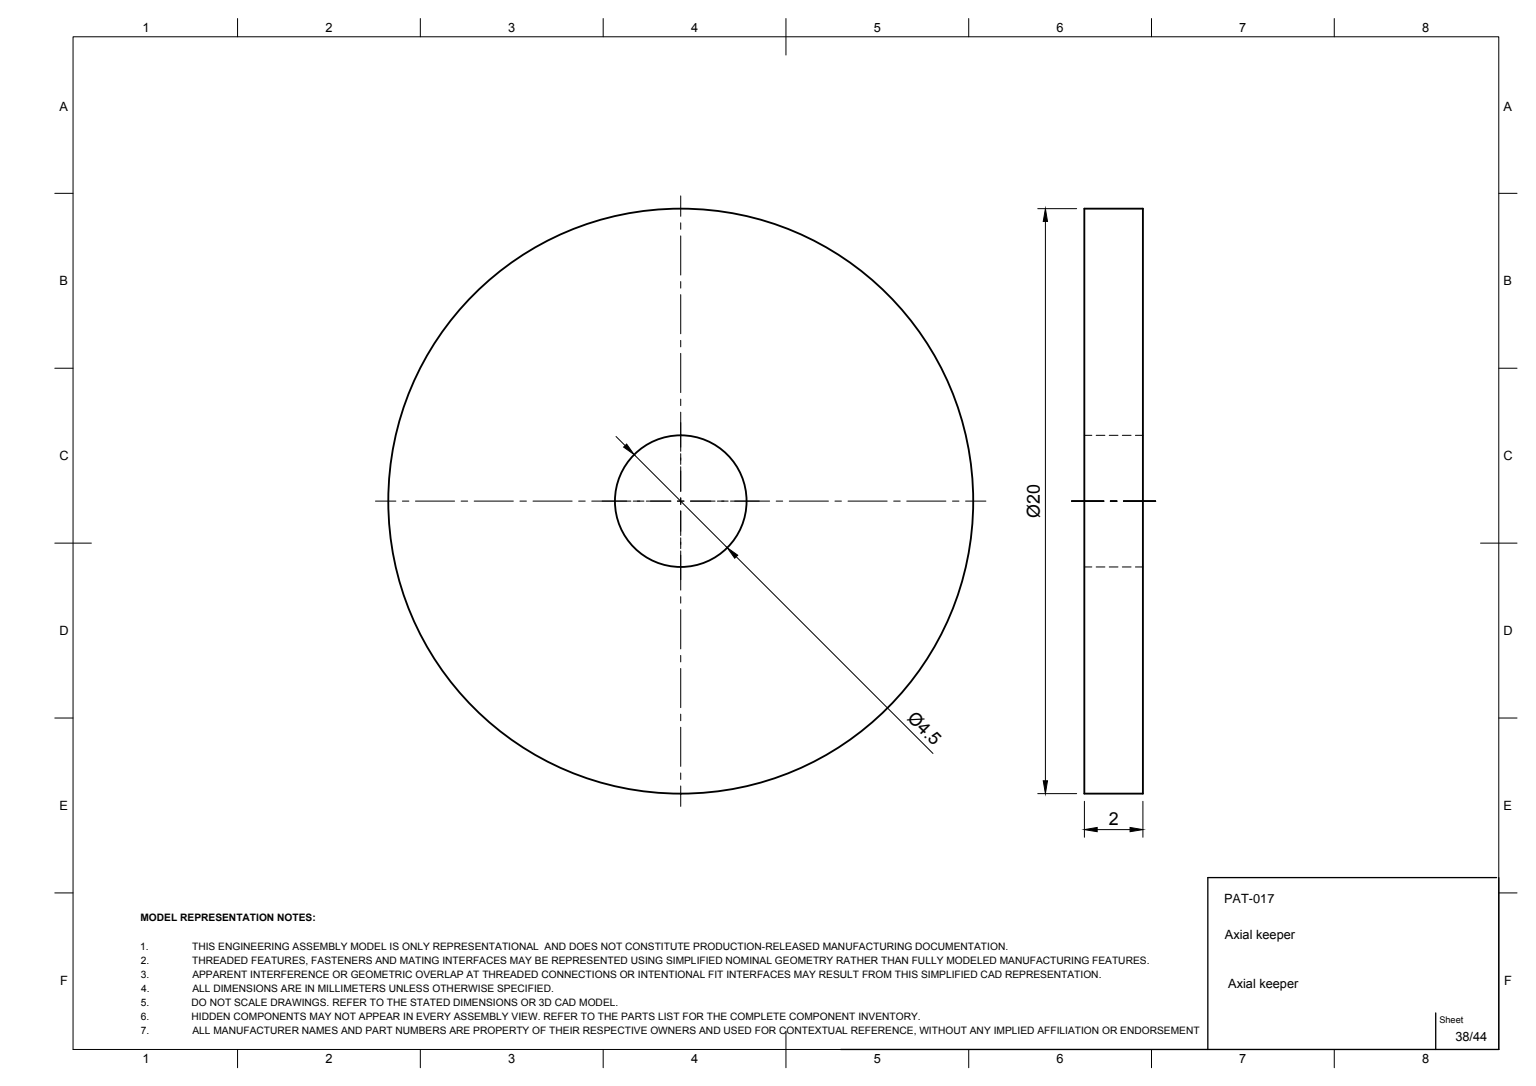
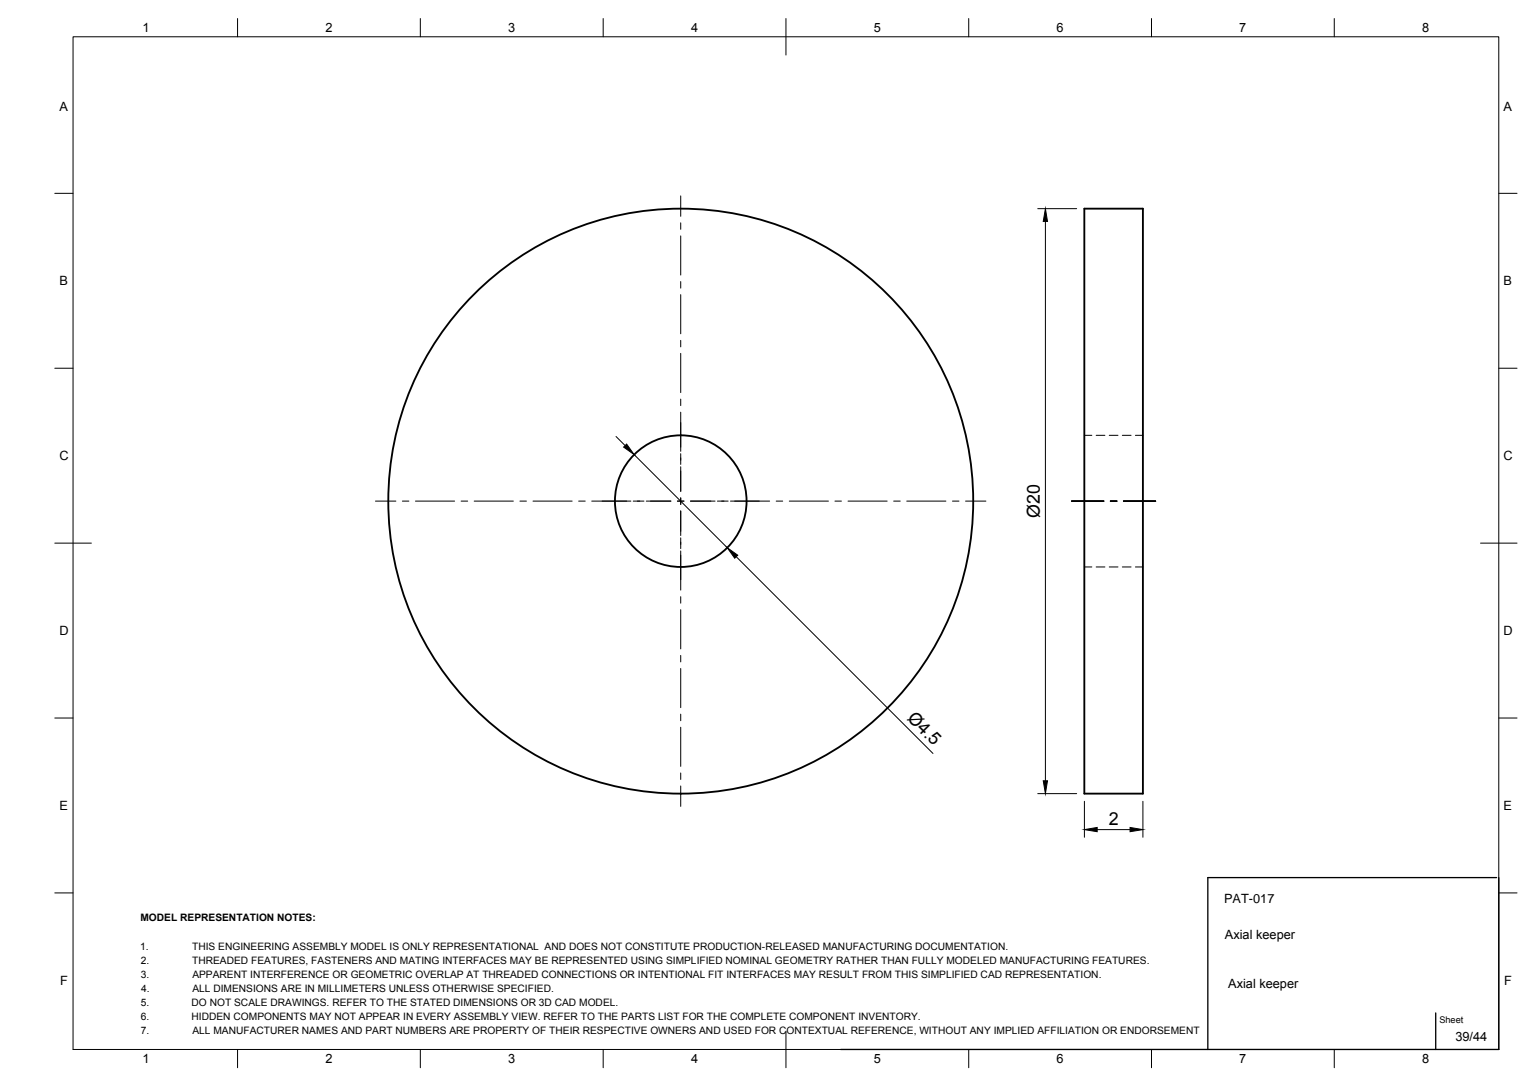
ISO-10303-21;
HEADER;
/* Generated by software containing ST-Developer
 * from STEP Tools, Inc. (www.steptools.com) 
 */

FILE_DESCRIPTION(
/* description */ ('Cam-and-follower valve demonstrator'),
/* implementation_level */ '2;1');

FILE_NAME(
/* name */ 'Axial keeper.step',
/* time_stamp */ '2026-10-28T03:25:17-07:00',
/* author */ (''),
/* organization */ (''),
/* preprocessor_version */ 'ST-DEVELOPER v20.2',
/* originating_system */ 'Autodesk Translation Framework v15.17.0.0',
/* authorisation */ '');

FILE_SCHEMA (('AUTOMOTIVE_DESIGN { 1 0 10303 214 3 1 1 }'));
ENDSEC;

DATA;
#10=MECHANICAL_DESIGN_GEOMETRIC_PRESENTATION_REPRESENTATION('',(#448),#12896);
#369=SHAPE_REPRESENTATION_RELATIONSHIP('SRR','None',#13088,#405);
#405=ADVANCED_BREP_SHAPE_REPRESENTATION('',(#489),#12888);
#448=STYLED_ITEM('',(#13316),#489);
#489=MANIFOLD_SOLID_BREP('Body1',#6217);
#648=FACE_BOUND('',#1934,.T.);
#649=FACE_BOUND('',#1936,.T.);
#945=CIRCLE('',#7265,0.225);
#946=CIRCLE('',#7266,0.225);
#947=CIRCLE('',#7268,1.);
#948=CIRCLE('',#7269,1.);
#1083=CYLINDRICAL_SURFACE('',#7264,0.225);
#1084=CYLINDRICAL_SURFACE('',#7267,1.);
#1410=FACE_OUTER_BOUND('',#1931,.T.);
#1411=FACE_OUTER_BOUND('',#1932,.T.);
#1412=FACE_OUTER_BOUND('',#1933,.T.);
#1413=FACE_OUTER_BOUND('',#1935,.T.);
#1931=EDGE_LOOP('',(#5401,#5402,#5403,#5404));
#1932=EDGE_LOOP('',(#5405,#5406,#5407,#5408));
#1933=EDGE_LOOP('',(#5409));
#1934=EDGE_LOOP('',(#5410));
#1935=EDGE_LOOP('',(#5411));
#1936=EDGE_LOOP('',(#5412));
#2347=LINE('',#12531,#2769);
#2348=LINE('',#12537,#2770);
#2769=VECTOR('',#9054,0.225);
#2770=VECTOR('',#9061,1.);
#3280=VERTEX_POINT('',#12528);
#3281=VERTEX_POINT('',#12530);
#3282=VERTEX_POINT('',#12534);
#3283=VERTEX_POINT('',#12536);
#3997=EDGE_CURVE('',#3280,#3280,#945,.T.);
#3998=EDGE_CURVE('',#3280,#3281,#2347,.T.);
#3999=EDGE_CURVE('',#3281,#3281,#946,.T.);
#4000=EDGE_CURVE('',#3282,#3282,#947,.T.);
#4001=EDGE_CURVE('',#3282,#3283,#2348,.T.);
#4002=EDGE_CURVE('',#3283,#3283,#948,.T.);
#5401=ORIENTED_EDGE('',*,*,#3997,.F.);
#5402=ORIENTED_EDGE('',*,*,#3998,.T.);
#5403=ORIENTED_EDGE('',*,*,#3999,.T.);
#5404=ORIENTED_EDGE('',*,*,#3998,.F.);
#5405=ORIENTED_EDGE('',*,*,#4000,.F.);
#5406=ORIENTED_EDGE('',*,*,#4001,.T.);
#5407=ORIENTED_EDGE('',*,*,#4002,.T.);
#5408=ORIENTED_EDGE('',*,*,#4001,.F.);
#5409=ORIENTED_EDGE('',*,*,#4000,.T.);
#5410=ORIENTED_EDGE('',*,*,#3997,.T.);
#5411=ORIENTED_EDGE('',*,*,#4002,.F.);
#5412=ORIENTED_EDGE('',*,*,#3999,.F.);
#5774=PLANE('',#7270);
#5775=PLANE('',#7271);
#6126=ADVANCED_FACE('',(#1410),#1083,.F.);
#6127=ADVANCED_FACE('',(#1411),#1084,.T.);
#6128=ADVANCED_FACE('',(#1412,#648),#5774,.T.);
#6129=ADVANCED_FACE('',(#1413,#649),#5775,.F.);
#6217=CLOSED_SHELL('',(#6126,#6127,#6128,#6129));
#7263=AXIS2_PLACEMENT_3D('',#12526,#9048,#9049);
#7264=AXIS2_PLACEMENT_3D('',#12527,#9050,#9051);
#7265=AXIS2_PLACEMENT_3D('',#12529,#9052,#9053);
#7266=AXIS2_PLACEMENT_3D('',#12532,#9055,#9056);
#7267=AXIS2_PLACEMENT_3D('',#12533,#9057,#9058);
#7268=AXIS2_PLACEMENT_3D('',#12535,#9059,#9060);
#7269=AXIS2_PLACEMENT_3D('',#12538,#9062,#9063);
#7270=AXIS2_PLACEMENT_3D('',#12539,#9064,#9065);
#7271=AXIS2_PLACEMENT_3D('',#12540,#9066,#9067);
#9048=DIRECTION('axis',(0.,0.,1.));
#9049=DIRECTION('refdir',(1.,0.,0.));
#9050=DIRECTION('center_axis',(0.,1.,0.));
#9051=DIRECTION('ref_axis',(1.,0.,0.));
#9052=DIRECTION('center_axis',(0.,-1.,0.));
#9053=DIRECTION('ref_axis',(1.,0.,0.));
#9054=DIRECTION('',(0.,-1.,0.));
#9055=DIRECTION('center_axis',(0.,-1.,0.));
#9056=DIRECTION('ref_axis',(1.,0.,0.));
#9057=DIRECTION('center_axis',(0.,1.,0.));
#9058=DIRECTION('ref_axis',(1.,0.,0.));
#9059=DIRECTION('center_axis',(0.,1.,0.));
#9060=DIRECTION('ref_axis',(1.,0.,0.));
#9061=DIRECTION('',(0.,-1.,0.));
#9062=DIRECTION('center_axis',(0.,1.,0.));
#9063=DIRECTION('ref_axis',(1.,0.,0.));
#9064=DIRECTION('center_axis',(0.,1.,0.));
#9065=DIRECTION('ref_axis',(1.,0.,0.));
#9066=DIRECTION('center_axis',(0.,1.,0.));
#9067=DIRECTION('ref_axis',(1.,0.,0.));
#12526=CARTESIAN_POINT('',(0.,0.,0.));
#12527=CARTESIAN_POINT('Origin',(0.,-4.7,4.));
#12528=CARTESIAN_POINT('',(-0.225,-4.5,4.));
#12529=CARTESIAN_POINT('Origin',(0.,-4.5,4.));
#12530=CARTESIAN_POINT('',(-0.225,-4.7,4.));
#12531=CARTESIAN_POINT('',(-0.225,-4.7,4.));
#12532=CARTESIAN_POINT('Origin',(0.,-4.7,4.));
#12533=CARTESIAN_POINT('Origin',(0.,-4.7,4.));
#12534=CARTESIAN_POINT('',(-1.,-4.5,4.));
#12535=CARTESIAN_POINT('Origin',(0.,-4.5,4.));
#12536=CARTESIAN_POINT('',(-1.,-4.7,4.));
#12537=CARTESIAN_POINT('',(-1.,-4.7,4.));
#12538=CARTESIAN_POINT('Origin',(0.,-4.7,4.));
#12539=CARTESIAN_POINT('Origin',(0.,-4.5,4.));
#12540=CARTESIAN_POINT('Origin',(0.,-4.7,4.));
#12845=UNCERTAINTY_MEASURE_WITH_UNIT(LENGTH_MEASURE(0.001),#12897,
'DISTANCE_ACCURACY_VALUE',
'Maximum model space distance between geometric entities at asserted c
onnectivities');
#12853=UNCERTAINTY_MEASURE_WITH_UNIT(LENGTH_MEASURE(0.001),#12897,
'DISTANCE_ACCURACY_VALUE',
'Maximum model space distance between geometric entities at asserted c
onnectivities');
#12888=(
GEOMETRIC_REPRESENTATION_CONTEXT(3)
GLOBAL_UNCERTAINTY_ASSIGNED_CONTEXT((#12845))
GLOBAL_UNIT_ASSIGNED_CONTEXT((#12897,#12899,#12900))
REPRESENTATION_CONTEXT('','3D')
);
#12896=(
GEOMETRIC_REPRESENTATION_CONTEXT(3)
GLOBAL_UNCERTAINTY_ASSIGNED_CONTEXT((#12853))
GLOBAL_UNIT_ASSIGNED_CONTEXT((#12897,#12899,#12900))
REPRESENTATION_CONTEXT('','3D')
);
#12897=(
LENGTH_UNIT()
NAMED_UNIT(*)
SI_UNIT(.CENTI.,.METRE.)
);
#12899=(
NAMED_UNIT(*)
PLANE_ANGLE_UNIT()
SI_UNIT($,.RADIAN.)
);
#12900=(
NAMED_UNIT(*)
SI_UNIT($,.STERADIAN.)
SOLID_ANGLE_UNIT()
);
#12935=SHAPE_DEFINITION_REPRESENTATION(#12984,#13088);
#12984=PRODUCT_DEFINITION_SHAPE('',$,#13131);
#13088=SHAPE_REPRESENTATION('',(#7263),#12888);
#13096=PRODUCT_DEFINITION_CONTEXT('part definition',#13224,'design');
#13131=PRODUCT_DEFINITION('Axial keeper','Axial keeper',#13173,#13096);
#13173=PRODUCT_DEFINITION_FORMATION('',$,#13260);
#13224=APPLICATION_CONTEXT(
'Core Data for Automotive Mechanical Design Process');
#13225=PRODUCT_CONTEXT('part definition',#13224,'mechanical');
#13260=PRODUCT('Axial keeper','Axial keeper','Axial keeper',(#13225));
#13310=COLOUR_RGB('Light Blue',0.38,0.62,0.78);
#13311=FILL_AREA_STYLE_COLOUR('',#13310);
#13312=FILL_AREA_STYLE('',(#13311));
#13313=SURFACE_STYLE_FILL_AREA(#13312);
#13314=SURFACE_SIDE_STYLE('',(#13313));
#13315=SURFACE_STYLE_USAGE(.BOTH.,#13314);
#13316=PRESENTATION_STYLE_ASSIGNMENT((#13315));
ENDSEC;
END-ISO-10303-21;
